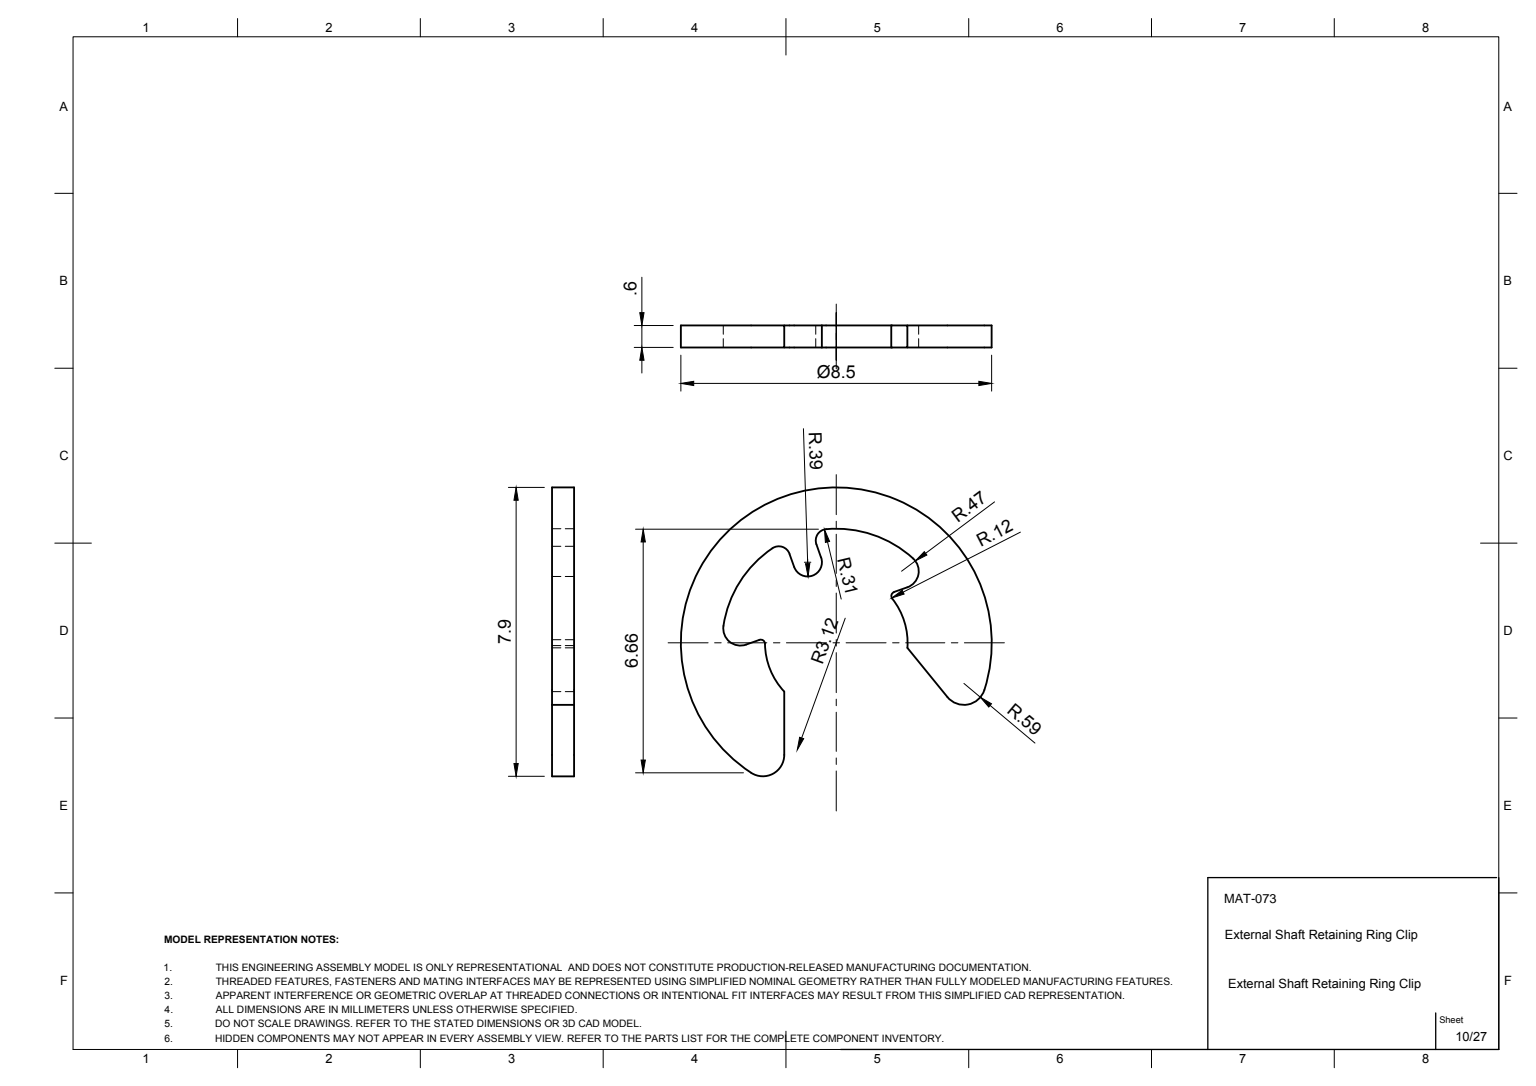
ISO-10303-21;
HEADER;
/* Generated by software containing ST-Developer
 * from STEP Tools, Inc. (www.steptools.com) 
 */

FILE_DESCRIPTION(
/* description */ ('CAx-IF Rec.Pracs.---Representation and Presentation of Product Manufa
cturing Information (PMI)---4.0---2014-10-13'),
/* implementation_level */ '2;1');

FILE_NAME(
/* name */ 'External Shaft Retaining Ring Clip.step',
/* time_stamp */ '2026-10-24T18:52:33-07:00',
/* author */ (''),
/* organization */ (''),
/* preprocessor_version */ 'ST-DEVELOPER v20.2',
/* originating_system */ 'Autodesk Translation Framework v15.17.0.0',
/* authorisation */ '');

FILE_SCHEMA (('AP242_MANAGED_MODEL_BASED_3D_ENGINEERING_MIM_LF { 1 0 10303 442 2 1 4 }'));
ENDSEC;

DATA;
#10=MECHANICAL_DESIGN_GEOMETRIC_PRESENTATION_REPRESENTATION('',(#423),#34876);
#357=SHAPE_REPRESENTATION_RELATIONSHIP('SRR','None',#34994,#390);
#390=ADVANCED_BREP_SHAPE_REPRESENTATION('',(#456),#34852);
#423=STYLED_ITEM('',(#35159),#456);
#456=MANIFOLD_SOLID_BREP('External Shaft Retaining Ring Clip',#19563);
#794=PLANE('',#20840);
#795=PLANE('',#20847);
#796=PLANE('',#20857);
#797=PLANE('',#20861);
#798=PLANE('',#20871);
#799=PLANE('',#20878);
#800=PLANE('',#20882);
#801=PLANE('',#20883);
#1677=LINE('',#30984,#3276);
#1678=LINE('',#30987,#3277);
#1679=LINE('',#30992,#3278);
#1680=LINE('',#30996,#3279);
#1681=LINE('',#30998,#3280);
#1682=LINE('',#30999,#3281);
#1683=LINE('',#31004,#3282);
#1684=LINE('',#31010,#3283);
#1685=LINE('',#31014,#3284);
#1686=LINE('',#31016,#3285);
#1687=LINE('',#31017,#3286);
#1688=LINE('',#31022,#3287);
#1689=LINE('',#31028,#3288);
#1690=LINE('',#31034,#3289);
#1691=LINE('',#31038,#3290);
#1692=LINE('',#31040,#3291);
#1693=LINE('',#31041,#3292);
#1694=LINE('',#31046,#3293);
#1695=LINE('',#31050,#3294);
#1696=LINE('',#31052,#3295);
#1697=LINE('',#31053,#3296);
#1698=LINE('',#31058,#3297);
#1699=LINE('',#31064,#3298);
#1700=LINE('',#31070,#3299);
#1701=LINE('',#31074,#3300);
#1702=LINE('',#31076,#3301);
#1703=LINE('',#31077,#3302);
#1704=LINE('',#31082,#3303);
#1705=LINE('',#31088,#3304);
#1706=LINE('',#31092,#3305);
#1707=LINE('',#31094,#3306);
#1708=LINE('',#31095,#3307);
#3276=VECTOR('',#24622,1.);
#3277=VECTOR('',#24625,1.);
#3278=VECTOR('',#24630,1.);
#3279=VECTOR('',#24635,1.);
#3280=VECTOR('',#24636,1.);
#3281=VECTOR('',#24637,1.);
#3282=VECTOR('',#24642,1.);
#3283=VECTOR('',#24649,1.);
#3284=VECTOR('',#24654,1.);
#3285=VECTOR('',#24655,1.);
#3286=VECTOR('',#24656,1.);
#3287=VECTOR('',#24661,1.);
#3288=VECTOR('',#24668,1.);
#3289=VECTOR('',#24675,1.);
#3290=VECTOR('',#24680,1.);
#3291=VECTOR('',#24681,1.);
#3292=VECTOR('',#24682,1.);
#3293=VECTOR('',#24687,1.);
#3294=VECTOR('',#24692,1.);
#3295=VECTOR('',#24693,1.);
#3296=VECTOR('',#24694,1.);
#3297=VECTOR('',#24699,1.);
#3298=VECTOR('',#24706,1.);
#3299=VECTOR('',#24713,1.);
#3300=VECTOR('',#24718,1.);
#3301=VECTOR('',#24719,1.);
#3302=VECTOR('',#24720,1.);
#3303=VECTOR('',#24725,1.);
#3304=VECTOR('',#24732,1.);
#3305=VECTOR('',#24737,1.);
#3306=VECTOR('',#24738,1.);
#3307=VECTOR('',#24739,1.);
#4468=CYLINDRICAL_SURFACE('',#20834,0.00425);
#4469=CYLINDRICAL_SURFACE('',#20837,0.000585);
#4470=CYLINDRICAL_SURFACE('',#20841,0.00195);
#4471=CYLINDRICAL_SURFACE('',#20844,0.000117);
#4472=CYLINDRICAL_SURFACE('',#20848,0.000468);
#4473=CYLINDRICAL_SURFACE('',#20851,0.00312);
#4474=CYLINDRICAL_SURFACE('',#20854,0.000312);
#4475=CYLINDRICAL_SURFACE('',#20858,0.00039);
#4476=CYLINDRICAL_SURFACE('',#20862,0.000312);
#4477=CYLINDRICAL_SURFACE('',#20865,0.00312);
#4478=CYLINDRICAL_SURFACE('',#20868,0.000468);
#4479=CYLINDRICAL_SURFACE('',#20872,0.000117);
#4480=CYLINDRICAL_SURFACE('',#20875,0.00195);
#4481=CYLINDRICAL_SURFACE('',#20879,0.000585);
#5194=FACE_OUTER_BOUND('',#6278,.T.);
#5195=FACE_OUTER_BOUND('',#6279,.T.);
#5196=FACE_OUTER_BOUND('',#6280,.T.);
#5197=FACE_OUTER_BOUND('',#6281,.T.);
#5198=FACE_OUTER_BOUND('',#6282,.T.);
#5199=FACE_OUTER_BOUND('',#6283,.T.);
#5200=FACE_OUTER_BOUND('',#6284,.T.);
#5201=FACE_OUTER_BOUND('',#6285,.T.);
#5202=FACE_OUTER_BOUND('',#6286,.T.);
#5203=FACE_OUTER_BOUND('',#6287,.T.);
#5204=FACE_OUTER_BOUND('',#6288,.T.);
#5205=FACE_OUTER_BOUND('',#6289,.T.);
#5206=FACE_OUTER_BOUND('',#6290,.T.);
#5207=FACE_OUTER_BOUND('',#6291,.T.);
#5208=FACE_OUTER_BOUND('',#6292,.T.);
#5209=FACE_OUTER_BOUND('',#6293,.T.);
#5210=FACE_OUTER_BOUND('',#6294,.T.);
#5211=FACE_OUTER_BOUND('',#6295,.T.);
#5212=FACE_OUTER_BOUND('',#6296,.T.);
#5213=FACE_OUTER_BOUND('',#6297,.T.);
#5214=FACE_OUTER_BOUND('',#6298,.T.);
#5215=FACE_OUTER_BOUND('',#6299,.T.);
#6278=EDGE_LOOP('',(#14976,#14977,#14978,#14979));
#6279=EDGE_LOOP('',(#14980,#14981,#14982,#14983));
#6280=EDGE_LOOP('',(#14984,#14985,#14986,#14987));
#6281=EDGE_LOOP('',(#14988,#14989,#14990,#14991));
#6282=EDGE_LOOP('',(#14992,#14993,#14994,#14995));
#6283=EDGE_LOOP('',(#14996,#14997,#14998,#14999));
#6284=EDGE_LOOP('',(#15000,#15001,#15002,#15003));
#6285=EDGE_LOOP('',(#15004,#15005,#15006,#15007));
#6286=EDGE_LOOP('',(#15008,#15009,#15010,#15011));
#6287=EDGE_LOOP('',(#15012,#15013,#15014,#15015));
#6288=EDGE_LOOP('',(#15016,#15017,#15018,#15019));
#6289=EDGE_LOOP('',(#15020,#15021,#15022,#15023));
#6290=EDGE_LOOP('',(#15024,#15025,#15026,#15027));
#6291=EDGE_LOOP('',(#15028,#15029,#15030,#15031));
#6292=EDGE_LOOP('',(#15032,#15033,#15034,#15035));
#6293=EDGE_LOOP('',(#15036,#15037,#15038,#15039));
#6294=EDGE_LOOP('',(#15040,#15041,#15042,#15043));
#6295=EDGE_LOOP('',(#15044,#15045,#15046,#15047));
#6296=EDGE_LOOP('',(#15048,#15049,#15050,#15051));
#6297=EDGE_LOOP('',(#15052,#15053,#15054,#15055));
#6298=EDGE_LOOP('',(#15056,#15057,#15058,#15059,#15060,#15061,#15062,#15063,
#15064,#15065,#15066,#15067,#15068,#15069,#15070,#15071,#15072,#15073,#15074,
#15075));
#6299=EDGE_LOOP('',(#15076,#15077,#15078,#15079,#15080,#15081,#15082,#15083,
#15084,#15085,#15086,#15087,#15088,#15089,#15090,#15091,#15092,#15093,#15094,
#15095));
#7376=CIRCLE('',#20835,0.00425000000001401);
#7377=CIRCLE('',#20836,0.00425000000001401);
#7378=CIRCLE('',#20838,0.000585000000012771);
#7379=CIRCLE('',#20839,0.000585000000012771);
#7380=CIRCLE('',#20842,0.00195000000001316);
#7381=CIRCLE('',#20843,0.00195000000001316);
#7382=CIRCLE('',#20845,0.00011700000001);
#7383=CIRCLE('',#20846,0.00011700000001);
#7384=CIRCLE('',#20849,0.00046800000001);
#7385=CIRCLE('',#20850,0.00046800000001);
#7386=CIRCLE('',#20852,0.00312000000001353);
#7387=CIRCLE('',#20853,0.00312000000001353);
#7388=CIRCLE('',#20855,0.000312000000012182);
#7389=CIRCLE('',#20856,0.000312000000012182);
#7390=CIRCLE('',#20859,0.00039000000001);
#7391=CIRCLE('',#20860,0.00039000000001);
#7392=CIRCLE('',#20863,0.00031200000001);
#7393=CIRCLE('',#20864,0.00031200000001);
#7394=CIRCLE('',#20866,0.00312000000001219);
#7395=CIRCLE('',#20867,0.00312000000001219);
#7396=CIRCLE('',#20869,0.00046800000001353);
#7397=CIRCLE('',#20870,0.00046800000001353);
#7398=CIRCLE('',#20873,0.000117000000012679);
#7399=CIRCLE('',#20874,0.000117000000012679);
#7400=CIRCLE('',#20876,0.00195000000001268);
#7401=CIRCLE('',#20877,0.00195000000001268);
#7402=CIRCLE('',#20880,0.000585000000014012);
#7403=CIRCLE('',#20881,0.000585000000014012);
#8792=VERTEX_POINT('',#30980);
#8793=VERTEX_POINT('',#30981);
#8794=VERTEX_POINT('',#30983);
#8795=VERTEX_POINT('',#30985);
#8796=VERTEX_POINT('',#30989);
#8797=VERTEX_POINT('',#30991);
#8798=VERTEX_POINT('',#30995);
#8799=VERTEX_POINT('',#30997);
#8800=VERTEX_POINT('',#31001);
#8801=VERTEX_POINT('',#31003);
#8802=VERTEX_POINT('',#31007);
#8803=VERTEX_POINT('',#31009);
#8804=VERTEX_POINT('',#31013);
#8805=VERTEX_POINT('',#31015);
#8806=VERTEX_POINT('',#31019);
#8807=VERTEX_POINT('',#31021);
#8808=VERTEX_POINT('',#31025);
#8809=VERTEX_POINT('',#31027);
#8810=VERTEX_POINT('',#31031);
#8811=VERTEX_POINT('',#31033);
#8812=VERTEX_POINT('',#31037);
#8813=VERTEX_POINT('',#31039);
#8814=VERTEX_POINT('',#31043);
#8815=VERTEX_POINT('',#31045);
#8816=VERTEX_POINT('',#31049);
#8817=VERTEX_POINT('',#31051);
#8818=VERTEX_POINT('',#31055);
#8819=VERTEX_POINT('',#31057);
#8820=VERTEX_POINT('',#31061);
#8821=VERTEX_POINT('',#31063);
#8822=VERTEX_POINT('',#31067);
#8823=VERTEX_POINT('',#31069);
#8824=VERTEX_POINT('',#31073);
#8825=VERTEX_POINT('',#31075);
#8826=VERTEX_POINT('',#31079);
#8827=VERTEX_POINT('',#31081);
#8828=VERTEX_POINT('',#31085);
#8829=VERTEX_POINT('',#31087);
#8830=VERTEX_POINT('',#31091);
#8831=VERTEX_POINT('',#31093);
#11046=EDGE_CURVE('',#8792,#8793,#7376,.T.);
#11047=EDGE_CURVE('',#8794,#8793,#1677,.T.);
#11048=EDGE_CURVE('',#8794,#8795,#7377,.T.);
#11049=EDGE_CURVE('',#8795,#8792,#1678,.T.);
#11050=EDGE_CURVE('',#8793,#8796,#7378,.T.);
#11051=EDGE_CURVE('',#8797,#8796,#1679,.T.);
#11052=EDGE_CURVE('',#8797,#8794,#7379,.T.);
#11053=EDGE_CURVE('',#8796,#8798,#1680,.T.);
#11054=EDGE_CURVE('',#8799,#8798,#1681,.T.);
#11055=EDGE_CURVE('',#8799,#8797,#1682,.T.);
#11056=EDGE_CURVE('',#8798,#8800,#7380,.T.);
#11057=EDGE_CURVE('',#8801,#8800,#1683,.T.);
#11058=EDGE_CURVE('',#8801,#8799,#7381,.T.);
#11059=EDGE_CURVE('',#8800,#8802,#7382,.T.);
#11060=EDGE_CURVE('',#8803,#8802,#1684,.T.);
#11061=EDGE_CURVE('',#8803,#8801,#7383,.T.);
#11062=EDGE_CURVE('',#8802,#8804,#1685,.T.);
#11063=EDGE_CURVE('',#8805,#8804,#1686,.T.);
#11064=EDGE_CURVE('',#8805,#8803,#1687,.T.);
#11065=EDGE_CURVE('',#8804,#8806,#7384,.T.);
#11066=EDGE_CURVE('',#8807,#8806,#1688,.T.);
#11067=EDGE_CURVE('',#8807,#8805,#7385,.T.);
#11068=EDGE_CURVE('',#8806,#8808,#7386,.T.);
#11069=EDGE_CURVE('',#8809,#8808,#1689,.T.);
#11070=EDGE_CURVE('',#8809,#8807,#7387,.T.);
#11071=EDGE_CURVE('',#8808,#8810,#7388,.T.);
#11072=EDGE_CURVE('',#8811,#8810,#1690,.T.);
#11073=EDGE_CURVE('',#8811,#8809,#7389,.T.);
#11074=EDGE_CURVE('',#8810,#8812,#1691,.T.);
#11075=EDGE_CURVE('',#8813,#8812,#1692,.T.);
#11076=EDGE_CURVE('',#8813,#8811,#1693,.T.);
#11077=EDGE_CURVE('',#8812,#8814,#7390,.T.);
#11078=EDGE_CURVE('',#8815,#8814,#1694,.T.);
#11079=EDGE_CURVE('',#8815,#8813,#7391,.T.);
#11080=EDGE_CURVE('',#8814,#8816,#1695,.T.);
#11081=EDGE_CURVE('',#8817,#8816,#1696,.T.);
#11082=EDGE_CURVE('',#8817,#8815,#1697,.T.);
#11083=EDGE_CURVE('',#8816,#8818,#7392,.T.);
#11084=EDGE_CURVE('',#8819,#8818,#1698,.T.);
#11085=EDGE_CURVE('',#8819,#8817,#7393,.T.);
#11086=EDGE_CURVE('',#8818,#8820,#7394,.T.);
#11087=EDGE_CURVE('',#8821,#8820,#1699,.T.);
#11088=EDGE_CURVE('',#8821,#8819,#7395,.T.);
#11089=EDGE_CURVE('',#8820,#8822,#7396,.T.);
#11090=EDGE_CURVE('',#8823,#8822,#1700,.T.);
#11091=EDGE_CURVE('',#8823,#8821,#7397,.T.);
#11092=EDGE_CURVE('',#8822,#8824,#1701,.T.);
#11093=EDGE_CURVE('',#8825,#8824,#1702,.T.);
#11094=EDGE_CURVE('',#8825,#8823,#1703,.T.);
#11095=EDGE_CURVE('',#8824,#8826,#7398,.T.);
#11096=EDGE_CURVE('',#8827,#8826,#1704,.T.);
#11097=EDGE_CURVE('',#8827,#8825,#7399,.T.);
#11098=EDGE_CURVE('',#8826,#8828,#7400,.T.);
#11099=EDGE_CURVE('',#8829,#8828,#1705,.T.);
#11100=EDGE_CURVE('',#8829,#8827,#7401,.T.);
#11101=EDGE_CURVE('',#8828,#8830,#1706,.T.);
#11102=EDGE_CURVE('',#8831,#8830,#1707,.T.);
#11103=EDGE_CURVE('',#8831,#8829,#1708,.T.);
#11104=EDGE_CURVE('',#8830,#8792,#7402,.T.);
#11105=EDGE_CURVE('',#8795,#8831,#7403,.T.);
#14976=ORIENTED_EDGE('',*,*,#11046,.T.);
#14977=ORIENTED_EDGE('',*,*,#11047,.F.);
#14978=ORIENTED_EDGE('',*,*,#11048,.T.);
#14979=ORIENTED_EDGE('',*,*,#11049,.T.);
#14980=ORIENTED_EDGE('',*,*,#11050,.T.);
#14981=ORIENTED_EDGE('',*,*,#11051,.F.);
#14982=ORIENTED_EDGE('',*,*,#11052,.T.);
#14983=ORIENTED_EDGE('',*,*,#11047,.T.);
#14984=ORIENTED_EDGE('',*,*,#11053,.T.);
#14985=ORIENTED_EDGE('',*,*,#11054,.F.);
#14986=ORIENTED_EDGE('',*,*,#11055,.T.);
#14987=ORIENTED_EDGE('',*,*,#11051,.T.);
#14988=ORIENTED_EDGE('',*,*,#11056,.T.);
#14989=ORIENTED_EDGE('',*,*,#11057,.F.);
#14990=ORIENTED_EDGE('',*,*,#11058,.T.);
#14991=ORIENTED_EDGE('',*,*,#11054,.T.);
#14992=ORIENTED_EDGE('',*,*,#11059,.T.);
#14993=ORIENTED_EDGE('',*,*,#11060,.F.);
#14994=ORIENTED_EDGE('',*,*,#11061,.T.);
#14995=ORIENTED_EDGE('',*,*,#11057,.T.);
#14996=ORIENTED_EDGE('',*,*,#11062,.T.);
#14997=ORIENTED_EDGE('',*,*,#11063,.F.);
#14998=ORIENTED_EDGE('',*,*,#11064,.T.);
#14999=ORIENTED_EDGE('',*,*,#11060,.T.);
#15000=ORIENTED_EDGE('',*,*,#11065,.T.);
#15001=ORIENTED_EDGE('',*,*,#11066,.F.);
#15002=ORIENTED_EDGE('',*,*,#11067,.T.);
#15003=ORIENTED_EDGE('',*,*,#11063,.T.);
#15004=ORIENTED_EDGE('',*,*,#11068,.T.);
#15005=ORIENTED_EDGE('',*,*,#11069,.F.);
#15006=ORIENTED_EDGE('',*,*,#11070,.T.);
#15007=ORIENTED_EDGE('',*,*,#11066,.T.);
#15008=ORIENTED_EDGE('',*,*,#11071,.T.);
#15009=ORIENTED_EDGE('',*,*,#11072,.F.);
#15010=ORIENTED_EDGE('',*,*,#11073,.T.);
#15011=ORIENTED_EDGE('',*,*,#11069,.T.);
#15012=ORIENTED_EDGE('',*,*,#11074,.T.);
#15013=ORIENTED_EDGE('',*,*,#11075,.F.);
#15014=ORIENTED_EDGE('',*,*,#11076,.T.);
#15015=ORIENTED_EDGE('',*,*,#11072,.T.);
#15016=ORIENTED_EDGE('',*,*,#11077,.T.);
#15017=ORIENTED_EDGE('',*,*,#11078,.F.);
#15018=ORIENTED_EDGE('',*,*,#11079,.T.);
#15019=ORIENTED_EDGE('',*,*,#11075,.T.);
#15020=ORIENTED_EDGE('',*,*,#11080,.T.);
#15021=ORIENTED_EDGE('',*,*,#11081,.F.);
#15022=ORIENTED_EDGE('',*,*,#11082,.T.);
#15023=ORIENTED_EDGE('',*,*,#11078,.T.);
#15024=ORIENTED_EDGE('',*,*,#11083,.T.);
#15025=ORIENTED_EDGE('',*,*,#11084,.F.);
#15026=ORIENTED_EDGE('',*,*,#11085,.T.);
#15027=ORIENTED_EDGE('',*,*,#11081,.T.);
#15028=ORIENTED_EDGE('',*,*,#11086,.T.);
#15029=ORIENTED_EDGE('',*,*,#11087,.F.);
#15030=ORIENTED_EDGE('',*,*,#11088,.T.);
#15031=ORIENTED_EDGE('',*,*,#11084,.T.);
#15032=ORIENTED_EDGE('',*,*,#11089,.T.);
#15033=ORIENTED_EDGE('',*,*,#11090,.F.);
#15034=ORIENTED_EDGE('',*,*,#11091,.T.);
#15035=ORIENTED_EDGE('',*,*,#11087,.T.);
#15036=ORIENTED_EDGE('',*,*,#11092,.T.);
#15037=ORIENTED_EDGE('',*,*,#11093,.F.);
#15038=ORIENTED_EDGE('',*,*,#11094,.T.);
#15039=ORIENTED_EDGE('',*,*,#11090,.T.);
#15040=ORIENTED_EDGE('',*,*,#11095,.T.);
#15041=ORIENTED_EDGE('',*,*,#11096,.F.);
#15042=ORIENTED_EDGE('',*,*,#11097,.T.);
#15043=ORIENTED_EDGE('',*,*,#11093,.T.);
#15044=ORIENTED_EDGE('',*,*,#11098,.T.);
#15045=ORIENTED_EDGE('',*,*,#11099,.F.);
#15046=ORIENTED_EDGE('',*,*,#11100,.T.);
#15047=ORIENTED_EDGE('',*,*,#11096,.T.);
#15048=ORIENTED_EDGE('',*,*,#11101,.T.);
#15049=ORIENTED_EDGE('',*,*,#11102,.F.);
#15050=ORIENTED_EDGE('',*,*,#11103,.T.);
#15051=ORIENTED_EDGE('',*,*,#11099,.T.);
#15052=ORIENTED_EDGE('',*,*,#11104,.T.);
#15053=ORIENTED_EDGE('',*,*,#11049,.F.);
#15054=ORIENTED_EDGE('',*,*,#11105,.T.);
#15055=ORIENTED_EDGE('',*,*,#11102,.T.);
#15056=ORIENTED_EDGE('',*,*,#11048,.F.);
#15057=ORIENTED_EDGE('',*,*,#11052,.F.);
#15058=ORIENTED_EDGE('',*,*,#11055,.F.);
#15059=ORIENTED_EDGE('',*,*,#11058,.F.);
#15060=ORIENTED_EDGE('',*,*,#11061,.F.);
#15061=ORIENTED_EDGE('',*,*,#11064,.F.);
#15062=ORIENTED_EDGE('',*,*,#11067,.F.);
#15063=ORIENTED_EDGE('',*,*,#11070,.F.);
#15064=ORIENTED_EDGE('',*,*,#11073,.F.);
#15065=ORIENTED_EDGE('',*,*,#11076,.F.);
#15066=ORIENTED_EDGE('',*,*,#11079,.F.);
#15067=ORIENTED_EDGE('',*,*,#11082,.F.);
#15068=ORIENTED_EDGE('',*,*,#11085,.F.);
#15069=ORIENTED_EDGE('',*,*,#11088,.F.);
#15070=ORIENTED_EDGE('',*,*,#11091,.F.);
#15071=ORIENTED_EDGE('',*,*,#11094,.F.);
#15072=ORIENTED_EDGE('',*,*,#11097,.F.);
#15073=ORIENTED_EDGE('',*,*,#11100,.F.);
#15074=ORIENTED_EDGE('',*,*,#11103,.F.);
#15075=ORIENTED_EDGE('',*,*,#11105,.F.);
#15076=ORIENTED_EDGE('',*,*,#11046,.F.);
#15077=ORIENTED_EDGE('',*,*,#11104,.F.);
#15078=ORIENTED_EDGE('',*,*,#11101,.F.);
#15079=ORIENTED_EDGE('',*,*,#11098,.F.);
#15080=ORIENTED_EDGE('',*,*,#11095,.F.);
#15081=ORIENTED_EDGE('',*,*,#11092,.F.);
#15082=ORIENTED_EDGE('',*,*,#11089,.F.);
#15083=ORIENTED_EDGE('',*,*,#11086,.F.);
#15084=ORIENTED_EDGE('',*,*,#11083,.F.);
#15085=ORIENTED_EDGE('',*,*,#11080,.F.);
#15086=ORIENTED_EDGE('',*,*,#11077,.F.);
#15087=ORIENTED_EDGE('',*,*,#11074,.F.);
#15088=ORIENTED_EDGE('',*,*,#11071,.F.);
#15089=ORIENTED_EDGE('',*,*,#11068,.F.);
#15090=ORIENTED_EDGE('',*,*,#11065,.F.);
#15091=ORIENTED_EDGE('',*,*,#11062,.F.);
#15092=ORIENTED_EDGE('',*,*,#11059,.F.);
#15093=ORIENTED_EDGE('',*,*,#11056,.F.);
#15094=ORIENTED_EDGE('',*,*,#11053,.F.);
#15095=ORIENTED_EDGE('',*,*,#11050,.F.);
#18910=ADVANCED_FACE('',(#5194),#4468,.T.);
#18911=ADVANCED_FACE('',(#5195),#4469,.T.);
#18912=ADVANCED_FACE('',(#5196),#794,.T.);
#18913=ADVANCED_FACE('',(#5197),#4470,.F.);
#18914=ADVANCED_FACE('',(#5198),#4471,.T.);
#18915=ADVANCED_FACE('',(#5199),#795,.T.);
#18916=ADVANCED_FACE('',(#5200),#4472,.F.);
#18917=ADVANCED_FACE('',(#5201),#4473,.F.);
#18918=ADVANCED_FACE('',(#5202),#4474,.F.);
#18919=ADVANCED_FACE('',(#5203),#796,.T.);
#18920=ADVANCED_FACE('',(#5204),#4475,.T.);
#18921=ADVANCED_FACE('',(#5205),#797,.T.);
#18922=ADVANCED_FACE('',(#5206),#4476,.F.);
#18923=ADVANCED_FACE('',(#5207),#4477,.F.);
#18924=ADVANCED_FACE('',(#5208),#4478,.F.);
#18925=ADVANCED_FACE('',(#5209),#798,.T.);
#18926=ADVANCED_FACE('',(#5210),#4479,.T.);
#18927=ADVANCED_FACE('',(#5211),#4480,.F.);
#18928=ADVANCED_FACE('',(#5212),#799,.T.);
#18929=ADVANCED_FACE('',(#5213),#4481,.T.);
#18930=ADVANCED_FACE('',(#5214),#800,.F.);
#18931=ADVANCED_FACE('',(#5215),#801,.T.);
#19563=CLOSED_SHELL('',(#18910,#18911,#18912,#18913,#18914,#18915,#18916,
#18917,#18918,#18919,#18920,#18921,#18922,#18923,#18924,#18925,#18926,#18927,
#18928,#18929,#18930,#18931));
#20833=AXIS2_PLACEMENT_3D('',#30978,#24616,#24617);
#20834=AXIS2_PLACEMENT_3D('',#30979,#24618,#24619);
#20835=AXIS2_PLACEMENT_3D('',#30982,#24620,#24621);
#20836=AXIS2_PLACEMENT_3D('',#30986,#24623,#24624);
#20837=AXIS2_PLACEMENT_3D('',#30988,#24626,#24627);
#20838=AXIS2_PLACEMENT_3D('',#30990,#24628,#24629);
#20839=AXIS2_PLACEMENT_3D('',#30993,#24631,#24632);
#20840=AXIS2_PLACEMENT_3D('',#30994,#24633,#24634);
#20841=AXIS2_PLACEMENT_3D('',#31000,#24638,#24639);
#20842=AXIS2_PLACEMENT_3D('',#31002,#24640,#24641);
#20843=AXIS2_PLACEMENT_3D('',#31005,#24643,#24644);
#20844=AXIS2_PLACEMENT_3D('',#31006,#24645,#24646);
#20845=AXIS2_PLACEMENT_3D('',#31008,#24647,#24648);
#20846=AXIS2_PLACEMENT_3D('',#31011,#24650,#24651);
#20847=AXIS2_PLACEMENT_3D('',#31012,#24652,#24653);
#20848=AXIS2_PLACEMENT_3D('',#31018,#24657,#24658);
#20849=AXIS2_PLACEMENT_3D('',#31020,#24659,#24660);
#20850=AXIS2_PLACEMENT_3D('',#31023,#24662,#24663);
#20851=AXIS2_PLACEMENT_3D('',#31024,#24664,#24665);
#20852=AXIS2_PLACEMENT_3D('',#31026,#24666,#24667);
#20853=AXIS2_PLACEMENT_3D('',#31029,#24669,#24670);
#20854=AXIS2_PLACEMENT_3D('',#31030,#24671,#24672);
#20855=AXIS2_PLACEMENT_3D('',#31032,#24673,#24674);
#20856=AXIS2_PLACEMENT_3D('',#31035,#24676,#24677);
#20857=AXIS2_PLACEMENT_3D('',#31036,#24678,#24679);
#20858=AXIS2_PLACEMENT_3D('',#31042,#24683,#24684);
#20859=AXIS2_PLACEMENT_3D('',#31044,#24685,#24686);
#20860=AXIS2_PLACEMENT_3D('',#31047,#24688,#24689);
#20861=AXIS2_PLACEMENT_3D('',#31048,#24690,#24691);
#20862=AXIS2_PLACEMENT_3D('',#31054,#24695,#24696);
#20863=AXIS2_PLACEMENT_3D('',#31056,#24697,#24698);
#20864=AXIS2_PLACEMENT_3D('',#31059,#24700,#24701);
#20865=AXIS2_PLACEMENT_3D('',#31060,#24702,#24703);
#20866=AXIS2_PLACEMENT_3D('',#31062,#24704,#24705);
#20867=AXIS2_PLACEMENT_3D('',#31065,#24707,#24708);
#20868=AXIS2_PLACEMENT_3D('',#31066,#24709,#24710);
#20869=AXIS2_PLACEMENT_3D('',#31068,#24711,#24712);
#20870=AXIS2_PLACEMENT_3D('',#31071,#24714,#24715);
#20871=AXIS2_PLACEMENT_3D('',#31072,#24716,#24717);
#20872=AXIS2_PLACEMENT_3D('',#31078,#24721,#24722);
#20873=AXIS2_PLACEMENT_3D('',#31080,#24723,#24724);
#20874=AXIS2_PLACEMENT_3D('',#31083,#24726,#24727);
#20875=AXIS2_PLACEMENT_3D('',#31084,#24728,#24729);
#20876=AXIS2_PLACEMENT_3D('',#31086,#24730,#24731);
#20877=AXIS2_PLACEMENT_3D('',#31089,#24733,#24734);
#20878=AXIS2_PLACEMENT_3D('',#31090,#24735,#24736);
#20879=AXIS2_PLACEMENT_3D('',#31096,#24740,#24741);
#20880=AXIS2_PLACEMENT_3D('',#31097,#24742,#24743);
#20881=AXIS2_PLACEMENT_3D('',#31098,#24744,#24745);
#20882=AXIS2_PLACEMENT_3D('',#31099,#24746,#24747);
#20883=AXIS2_PLACEMENT_3D('',#31100,#24748,#24749);
#24616=DIRECTION('axis',(0.,0.,1.));
#24617=DIRECTION('refdir',(1.,0.,0.));
#24618=DIRECTION('center_axis',(2.07638679158937E-16,-1.,1.20948400507518E-31));
#24619=DIRECTION('ref_axis',(0.00551570721125935,1.14527415997344E-18,0.999984788371283));
#24620=DIRECTION('center_axis',(-2.07638679158937E-16,1.,-1.20948400507518E-31));
#24621=DIRECTION('ref_axis',(0.792981602406797,1.64653652521085E-16,-0.609245581226774));
#24622=DIRECTION('',(2.07638679158937E-16,-1.,1.20948400507518E-31));
#24623=DIRECTION('center_axis',(2.07638679158937E-16,-1.,1.20948400507518E-31));
#24624=DIRECTION('ref_axis',(0.792981602406797,1.64653652521085E-16,-0.609245581226774));
#24625=DIRECTION('',(2.07638679158937E-16,-1.,1.20948400507518E-31));
#24626=DIRECTION('center_axis',(2.07638679158937E-16,-1.,1.20948400507518E-31));
#24627=DIRECTION('ref_axis',(-0.944120330982807,-1.96035898492368E-16,-0.329600971820345));
#24628=DIRECTION('center_axis',(-2.07638679158937E-16,1.,-1.20948400507518E-31));
#24629=DIRECTION('ref_axis',(-0.944120330979384,-1.96035898491658E-16,-0.329600971830149));
#24630=DIRECTION('',(2.07638679158937E-16,-1.,1.20948400507518E-31));
#24631=DIRECTION('center_axis',(2.07638679158937E-16,-1.,1.20948400507518E-31));
#24632=DIRECTION('ref_axis',(-0.944120330979384,-1.96035898491658E-16,-0.329600971830149));
#24633=DIRECTION('center_axis',(-0.944120330982807,-1.96035898492369E-16,
-0.329600971820345));
#24634=DIRECTION('ref_axis',(-0.329600971820345,-6.84379104382785E-17,0.944120330982807));
#24635=DIRECTION('',(-0.329600971820918,-6.84379104383976E-17,0.944120330982607));
#24636=DIRECTION('',(2.07638679158937E-16,-1.,1.20948400507518E-31));
#24637=DIRECTION('',(0.329600971820918,6.84379104383976E-17,-0.944120330982607));
#24638=DIRECTION('center_axis',(2.07638679158937E-16,-1.,1.20948400507518E-31));
#24639=DIRECTION('ref_axis',(-0.914294914418656,-1.89842988391623E-16,0.405049144509876));
#24640=DIRECTION('center_axis',(2.07638679158937E-16,-1.,1.20948400507518E-31));
#24641=DIRECTION('ref_axis',(-0.914294914417583,-1.898429883914E-16,0.405049144512298));
#24642=DIRECTION('',(2.07638679158937E-16,-1.,1.20948400507518E-31));
#24643=DIRECTION('center_axis',(-2.07638679158937E-16,1.,-1.20948400507518E-31));
#24644=DIRECTION('ref_axis',(-0.914294914417583,-1.898429883914E-16,0.405049144512298));
#24645=DIRECTION('center_axis',(2.07638679158937E-16,-1.,1.20948400507518E-31));
#24646=DIRECTION('ref_axis',(0.00551570721125941,1.14527415997345E-18,0.999984788371283));
#24647=DIRECTION('center_axis',(-2.07638679158937E-16,1.,-1.20948400507518E-31));
#24648=DIRECTION('ref_axis',(0.00551570721125941,1.14527415997345E-18,0.999984788371283));
#24649=DIRECTION('',(2.07638679158937E-16,-1.,1.20948400507518E-31));
#24650=DIRECTION('center_axis',(2.07638679158937E-16,-1.,1.20948400507518E-31));
#24651=DIRECTION('ref_axis',(0.00551570721125941,1.14527415997345E-18,0.999984788371283));
#24652=DIRECTION('center_axis',(0.00551570721125941,1.14527415997345E-18,
0.999984788371283));
#24653=DIRECTION('ref_axis',(0.999984788371283,2.07635520636443E-16,-0.00551570721125941));
#24654=DIRECTION('',(0.999984788371283,2.07635520636443E-16,-0.00551570721125941));
#24655=DIRECTION('',(2.07638679158937E-16,-1.,1.20948400507518E-31));
#24656=DIRECTION('',(-0.999984788371283,-2.07635520636443E-16,0.00551570721125941));
#24657=DIRECTION('center_axis',(2.07638679158937E-16,-1.,1.20948400507518E-31));
#24658=DIRECTION('ref_axis',(0.00551570721125941,1.14527415997345E-18,0.999984788371283));
#24659=DIRECTION('center_axis',(2.07638679158937E-16,-1.,1.20948400507518E-31));
#24660=DIRECTION('ref_axis',(0.00551570721125941,1.14527415997345E-18,0.999984788371283));
#24661=DIRECTION('',(2.07638679158937E-16,-1.,1.20948400507518E-31));
#24662=DIRECTION('center_axis',(-2.07638679158937E-16,1.,-1.20948400507518E-31));
#24663=DIRECTION('ref_axis',(0.00551570721125941,1.14527415997345E-18,0.999984788371283));
#24664=DIRECTION('center_axis',(2.07638679158937E-16,-1.,1.20948400507518E-31));
#24665=DIRECTION('ref_axis',(-0.884935146074078,-1.83746764872143E-16,-0.465714276400081));
#24666=DIRECTION('center_axis',(2.07638679158937E-16,-1.,1.20948400507518E-31));
#24667=DIRECTION('ref_axis',(-0.884935146073463,-1.83746764872015E-16,-0.465714276401249));
#24668=DIRECTION('',(2.07638679158937E-16,-1.,1.20948400507518E-31));
#24669=DIRECTION('center_axis',(-2.07638679158937E-16,1.,-1.20948400507518E-31));
#24670=DIRECTION('ref_axis',(-0.884935146073463,-1.83746764872015E-16,-0.465714276401249));
#24671=DIRECTION('center_axis',(2.07638679158937E-16,-1.,1.20948400507518E-31));
#24672=DIRECTION('ref_axis',(-0.255336757635762,-5.30177870962154E-17,-0.966852181152867));
#24673=DIRECTION('center_axis',(2.07638679158937E-16,-1.,1.20948400507518E-31));
#24674=DIRECTION('ref_axis',(-0.25533675765802,-5.3017787100837E-17,-0.966852181146989));
#24675=DIRECTION('',(2.07638679158937E-16,-1.,1.20948400507518E-31));
#24676=DIRECTION('center_axis',(-2.07638679158937E-16,1.,-1.20948400507518E-31));
#24677=DIRECTION('ref_axis',(-0.25533675765802,-5.3017787100837E-17,-0.966852181146989));
#24678=DIRECTION('center_axis',(0.999984788371283,2.07635520636443E-16,
-0.00551570721125978));
#24679=DIRECTION('ref_axis',(2.07638679158938E-16,-1.,1.17369458351054E-31));
#24680=DIRECTION('',(-0.00551570721225976,-1.14527416018116E-18,-0.999984788371277));
#24681=DIRECTION('',(2.07638679158937E-16,-1.,1.20948400507518E-31));
#24682=DIRECTION('',(0.00551570721225976,1.14527416018116E-18,0.999984788371277));
#24683=DIRECTION('center_axis',(2.07638679158937E-16,-1.,1.20948400507518E-31));
#24684=DIRECTION('ref_axis',(-0.999984788371283,-2.07635520636442E-16,0.00551570721125905));
#24685=DIRECTION('center_axis',(-2.07638679158937E-16,1.,-1.20948400507518E-31));
#24686=DIRECTION('ref_axis',(-0.999984788371424,-2.07635520636472E-16,0.00551570718561842));
#24687=DIRECTION('',(2.07638679158937E-16,-1.,1.20948400507518E-31));
#24688=DIRECTION('center_axis',(2.07638679158937E-16,-1.,1.20948400507518E-31));
#24689=DIRECTION('ref_axis',(-0.999984788371424,-2.07635520636472E-16,0.00551570718561842));
#24690=DIRECTION('center_axis',(-0.999984788371283,-2.07635520636443E-16,
0.00551570721125904));
#24691=DIRECTION('ref_axis',(0.00551570721125904,1.14527415997337E-18,0.999984788371283));
#24692=DIRECTION('',(0.00551570721025906,1.14527415976574E-18,0.999984788371289));
#24693=DIRECTION('',(2.07638679158937E-16,-1.,1.20948400507518E-31));
#24694=DIRECTION('',(-0.00551570721025906,-1.14527415976574E-18,-0.999984788371289));
#24695=DIRECTION('center_axis',(2.07638679158937E-16,-1.,1.20948400507518E-31));
#24696=DIRECTION('ref_axis',(-0.999984788371283,-2.07635520636442E-16,0.00551570721125908));
#24697=DIRECTION('center_axis',(2.07638679158937E-16,-1.,1.20948400507518E-31));
#24698=DIRECTION('ref_axis',(-0.99998478837146,-2.07635520636479E-16,0.00551570717920828));
#24699=DIRECTION('',(2.07638679158937E-16,-1.,1.20948400507518E-31));
#24700=DIRECTION('center_axis',(-2.07638679158937E-16,1.,-1.20948400507518E-31));
#24701=DIRECTION('ref_axis',(-0.99998478837146,-2.07635520636479E-16,0.00551570717920828));
#24702=DIRECTION('center_axis',(2.07638679158937E-16,-1.,1.20948400507518E-31));
#24703=DIRECTION('ref_axis',(0.24465563654988,5.07999732220059E-17,-0.969610034758496));
#24704=DIRECTION('center_axis',(2.07638679158937E-16,-1.,1.20948400507518E-31));
#24705=DIRECTION('ref_axis',(0.244655636552112,5.07999732224693E-17,-0.969610034757934));
#24706=DIRECTION('',(2.07638679158937E-16,-1.,1.20948400507518E-31));
#24707=DIRECTION('center_axis',(-2.07638679158937E-16,1.,-1.20948400507518E-31));
#24708=DIRECTION('ref_axis',(0.244655636552112,5.07999732224693E-17,-0.969610034757934));
#24709=DIRECTION('center_axis',(2.07638679158937E-16,-1.,1.20948400507518E-31));
#24710=DIRECTION('ref_axis',(0.879743892228186,1.82668859780403E-16,-0.475447877361127));
#24711=DIRECTION('center_axis',(2.07638679158937E-16,-1.,1.20948400507518E-31));
#24712=DIRECTION('ref_axis',(0.879743892224003,1.82668859779534E-16,-0.475447877368867));
#24713=DIRECTION('',(2.07638679158937E-16,-1.,1.20948400507518E-31));
#24714=DIRECTION('center_axis',(-2.07638679158937E-16,1.,-1.20948400507518E-31));
#24715=DIRECTION('ref_axis',(0.879743892224003,1.82668859779534E-16,-0.475447877368867));
#24716=DIRECTION('center_axis',(0.00551570721125941,1.14527415997345E-18,
0.999984788371283));
#24717=DIRECTION('ref_axis',(0.999984788371283,2.07635520636443E-16,-0.00551570721125941));
#24718=DIRECTION('',(0.999984788371283,2.07635520636443E-16,-0.00551570721125941));
#24719=DIRECTION('',(2.07638679158937E-16,-1.,1.20948400507518E-31));
#24720=DIRECTION('',(-0.999984788371283,-2.07635520636443E-16,0.00551570721125941));
#24721=DIRECTION('center_axis',(2.07638679158937E-16,-1.,1.20948400507518E-31));
#24722=DIRECTION('ref_axis',(0.945378697202868,1.962971839922E-16,-0.325974107675761));
#24723=DIRECTION('center_axis',(-2.07638679158937E-16,1.,-1.20948400507518E-31));
#24724=DIRECTION('ref_axis',(0.945378697185416,1.96297183988576E-16,-0.325974107726375));
#24725=DIRECTION('',(2.07638679158937E-16,-1.,1.20948400507518E-31));
#24726=DIRECTION('center_axis',(2.07638679158937E-16,-1.,1.20948400507518E-31));
#24727=DIRECTION('ref_axis',(0.945378697185416,1.96297183988576E-16,-0.325974107726375));
#24728=DIRECTION('center_axis',(2.07638679158937E-16,-1.,1.20948400507518E-31));
#24729=DIRECTION('ref_axis',(0.945378697202867,1.962971839922E-16,-0.325974107675763));
#24730=DIRECTION('center_axis',(2.07638679158937E-16,-1.,1.20948400507518E-31));
#24731=DIRECTION('ref_axis',(0.94537869720182,1.96297183991983E-16,-0.3259741076788));
#24732=DIRECTION('',(2.07638679158937E-16,-1.,1.20948400507518E-31));
#24733=DIRECTION('center_axis',(-2.07638679158937E-16,1.,-1.20948400507518E-31));
#24734=DIRECTION('ref_axis',(0.94537869720182,1.96297183991983E-16,-0.3259741076788));
#24735=DIRECTION('center_axis',(0.94042697538271,1.952690150139E-16,-0.339995741109396));
#24736=DIRECTION('ref_axis',(-2.07638679158937E-16,1.,-1.30537451319996E-31));
#24737=DIRECTION('',(-0.339995741109967,-7.05962666037377E-17,-0.940426975382504));
#24738=DIRECTION('',(2.07638679158937E-16,-1.,1.20948400507518E-31));
#24739=DIRECTION('',(0.339995741109967,7.05962666037377E-17,0.940426975382504));
#24740=DIRECTION('center_axis',(2.07638679158937E-16,-1.,1.20948400507518E-31));
#24741=DIRECTION('ref_axis',(-0.799654090863859,-1.66039119211012E-16,-0.600460935419362));
#24742=DIRECTION('center_axis',(-2.07638679158937E-16,1.,-1.20948400507518E-31));
#24743=DIRECTION('ref_axis',(-0.799654090861894,-1.66039119210604E-16,-0.600460935421979));
#24744=DIRECTION('center_axis',(2.07638679158937E-16,-1.,1.20948400507518E-31));
#24745=DIRECTION('ref_axis',(-0.799654090861894,-1.66039119210604E-16,-0.600460935421979));
#24746=DIRECTION('center_axis',(2.07638679158937E-16,-1.,1.20948400507518E-31));
#24747=DIRECTION('ref_axis',(0.999984788371283,2.07635520636442E-16,-0.00551570721125941));
#24748=DIRECTION('center_axis',(2.07638679158937E-16,-1.,1.20948400507518E-31));
#24749=DIRECTION('ref_axis',(0.999984788371283,2.07635520636442E-16,-0.00551570721125941));
#30978=CARTESIAN_POINT('',(0.,0.,0.));
#30979=CARTESIAN_POINT('Origin',(-4.35815392021282E-17,-0.02565,3.46944695195361E-18));
#30980=CARTESIAN_POINT('',(-0.00339852988617145,-0.02625,-0.00255195897553229));
#30981=CARTESIAN_POINT('',(0.00337017181023001,-0.02625,-0.00258929372021227));
#30982=CARTESIAN_POINT('Origin',(9.90123578286685E-15,-0.02625000000001,
-1.00514215006786E-14));
#30983=CARTESIAN_POINT('',(0.00337017181023001,-0.02565,-0.00258929372021227));
#30984=CARTESIAN_POINT('',(0.00337017181023996,-0.02565,-0.00258929372022232));
#30985=CARTESIAN_POINT('',(-0.00339852988617145,-0.02565,-0.00255195897553229));
#30986=CARTESIAN_POINT('Origin',(9.90111042199066E-15,-0.02565,-1.00514215006786E-14));
#30987=CARTESIAN_POINT('',(-0.0033985298861815,-0.02565,-0.00255195897554223));
#30988=CARTESIAN_POINT('Origin',(0.00290627757282187,-0.02565,-0.00223288505519481));
#30989=CARTESIAN_POINT('',(0.00235396717919693,-0.02625,-0.00242570162370972));
#30990=CARTESIAN_POINT('Origin',(0.00290627757283182,-0.02625000000001,
-0.00223288505520486));
#30991=CARTESIAN_POINT('',(0.00235396717919693,-0.02565,-0.00242570162370972));
#30992=CARTESIAN_POINT('',(0.00235396717920687,-0.02565,-0.00242570162371977));
#30993=CARTESIAN_POINT('Origin',(0.00290627757283182,-0.02565,-0.00223288505520486));
#30994=CARTESIAN_POINT('Origin',(0.00235396717919693,-0.02565,-0.00242570162370972));
#30995=CARTESIAN_POINT('',(0.00178287508311634,-0.02625,-0.000789845831794254));
#30996=CARTESIAN_POINT('',(0.00178287508312629,-0.02625000000001,-0.000789845831804309));
#30997=CARTESIAN_POINT('',(0.00178287508311634,-0.02565,-0.000789845831794254));
#30998=CARTESIAN_POINT('',(0.00178287508312629,-0.02565,-0.000789845831804309));
#30999=CARTESIAN_POINT('',(0.00178287508312629,-0.02565,-0.000789845831804309));
#31000=CARTESIAN_POINT('Origin',(-4.35815392021282E-17,-0.02565,3.46944695195361E-18));
#31001=CARTESIAN_POINT('',(0.00185038829705699,-0.02625,0.000615274857372195));
#31002=CARTESIAN_POINT('Origin',(9.90123578286685E-15,-0.02625000000001,
-1.00514215006786E-14));
#31003=CARTESIAN_POINT('',(0.00185038829705699,-0.02565,0.000615274857372195));
#31004=CARTESIAN_POINT('',(0.00185038829706693,-0.02565,0.00061527485736214));
#31005=CARTESIAN_POINT('Origin',(9.90111042199066E-15,-0.02565,-1.00514215006786E-14));
#31006=CARTESIAN_POINT('Origin',(0.00196141159488042,-0.02565,0.000652191348814524));
#31007=CARTESIAN_POINT('',(0.00196205693262413,-0.02625,0.000769189569053964));
#31008=CARTESIAN_POINT('Origin',(0.00196141159489036,-0.02625000000001,
0.000652191348804469));
#31009=CARTESIAN_POINT('',(0.00196205693262413,-0.02565,0.000769189569053964));
#31010=CARTESIAN_POINT('',(0.00196205693263408,-0.02565,0.000769189569043909));
#31011=CARTESIAN_POINT('Origin',(0.00196141159489036,-0.02565,0.000652191348804469));
#31012=CARTESIAN_POINT('Origin',(0.00196205693262413,-0.02565,0.000769189569053964));
#31013=CARTESIAN_POINT('',(0.00234426665641354,-0.02625,0.000767081380055257));
#31014=CARTESIAN_POINT('',(0.00234426665642348,-0.02625000000001,0.000767081380045202));
#31015=CARTESIAN_POINT('',(0.00234426665641354,-0.02565,0.000767081380055257));
#31016=CARTESIAN_POINT('',(0.00234426665642348,-0.02565,0.000767081380045202));
#31017=CARTESIAN_POINT('',(0.00234426665642348,-0.02565,0.000767081380045202));
#31018=CARTESIAN_POINT('Origin',(0.00234684800738841,-0.02565,0.00123507426101302));
#31019=CARTESIAN_POINT('',(0.00276099765575108,-0.02625,0.00145302854236826));
#31020=CARTESIAN_POINT('Origin',(0.00234684800739835,-0.02625000000001,
0.00123507426100296));
#31021=CARTESIAN_POINT('',(0.00276099765575108,-0.02565,0.00145302854236826));
#31022=CARTESIAN_POINT('',(0.00276099765576102,-0.02565,0.0014530285423582));
#31023=CARTESIAN_POINT('Origin',(0.00234684800739835,-0.02565,0.00123507426100296));
#31024=CARTESIAN_POINT('Origin',(-4.35815392021282E-17,-0.02565,3.46944695195361E-18));
#31025=CARTESIAN_POINT('',(0.000796650683823533,-0.02625,0.00301657880519694));
#31026=CARTESIAN_POINT('Origin',(9.90123578286685E-15,-0.02625000000001,
-1.00514215006786E-14));
#31027=CARTESIAN_POINT('',(0.000796650683823533,-0.02565,0.00301657880519694));
#31028=CARTESIAN_POINT('',(0.000796650683833588,-0.02565,0.00301657880520689));
#31029=CARTESIAN_POINT('Origin',(9.90111042199066E-15,-0.02565,-1.00514215006786E-14));
#31030=CARTESIAN_POINT('Origin',(0.000716985615441175,-0.02565,0.00271492092467725));
#31031=CARTESIAN_POINT('',(0.000404990361469335,-0.02625,0.00271664182532716));
#31032=CARTESIAN_POINT('Origin',(0.00071698561545123,-0.02625000000001,
0.0027149209246872));
#31033=CARTESIAN_POINT('',(0.000404990361469334,-0.02565,0.00271664182532716));
#31034=CARTESIAN_POINT('',(0.000404990361479389,-0.02565,0.00271664182533711));
#31035=CARTESIAN_POINT('Origin',(0.00071698561545123,-0.02565,0.0027149209246872));
#31036=CARTESIAN_POINT('Origin',(0.000404990361469334,-0.02565,0.00271664182532716));
#31037=CARTESIAN_POINT('',(0.000402900822339103,-0.02625,0.00233781327897642));
#31038=CARTESIAN_POINT('',(0.000402900822349048,-0.02625000000001,0.00233781327896636));
#31039=CARTESIAN_POINT('',(0.000402900822339103,-0.02565,0.00233781327897642));
#31040=CARTESIAN_POINT('',(0.000402900822349048,-0.02565,0.00233781327896636));
#31041=CARTESIAN_POINT('',(0.000402900822349048,-0.02565,0.00233781327896636));
#31042=CARTESIAN_POINT('Origin',(1.29067548743032E-5,-0.02565,0.00233996440478881));
#31043=CARTESIAN_POINT('',(-0.000377087312590497,-0.02625,0.0023421155306012));
#31044=CARTESIAN_POINT('Origin',(1.29067548742481E-5,-0.02625000000001,
0.00233996440477881));
#31045=CARTESIAN_POINT('',(-0.000377087312590497,-0.02565,0.0023421155306012));
#31046=CARTESIAN_POINT('',(-0.000377087312600552,-0.02565,0.00234211553059125));
#31047=CARTESIAN_POINT('Origin',(1.2906754874248E-5,-0.02565,0.00233996440477881));
#31048=CARTESIAN_POINT('Origin',(-0.000377087312590497,-0.02565,0.0023421155306012));
#31049=CARTESIAN_POINT('',(-0.000374997773460266,-0.02625,0.00272094407695195));
#31050=CARTESIAN_POINT('',(-0.000374997773470211,-0.02625000000001,0.00272094407696201));
#31051=CARTESIAN_POINT('',(-0.000374997773460266,-0.02565,0.00272094407695195));
#31052=CARTESIAN_POINT('',(-0.000374997773470211,-0.02565,0.00272094407696201));
#31053=CARTESIAN_POINT('',(-0.000374997773470211,-0.02565,0.00272094407696201));
#31054=CARTESIAN_POINT('Origin',(-0.000686993027432106,-0.02565,0.00272266497760186));
#31055=CARTESIAN_POINT('',(-0.000763325586035669,-0.02625,0.00302518330844651));
#31056=CARTESIAN_POINT('Origin',(-0.000686993027442051,-0.02625000000001,
0.00272266497761192));
#31057=CARTESIAN_POINT('',(-0.000763325586035669,-0.02565,0.00302518330844651));
#31058=CARTESIAN_POINT('',(-0.000763325586045614,-0.02565,0.00302518330845656));
#31059=CARTESIAN_POINT('Origin',(-0.000686993027442051,-0.02565,0.00272266497761192));
#31060=CARTESIAN_POINT('Origin',(-4.35815392021282E-17,-0.02565,3.46944695195361E-18));
#31061=CARTESIAN_POINT('',(-0.00274480094375199,-0.02625,0.00148339737736672));
#31062=CARTESIAN_POINT('Origin',(9.90123578286685E-15,-0.02625000000001,
-1.00514215006786E-14));
#31063=CARTESIAN_POINT('',(-0.00274480094375199,-0.02565,0.00148339737736672));
#31064=CARTESIAN_POINT('',(-0.00274480094376204,-0.02565,0.00148339737735678));
#31065=CARTESIAN_POINT('Origin',(9.90111042199066E-15,-0.02565,-1.00514215006786E-14));
#31066=CARTESIAN_POINT('Origin',(-0.00233308080218919,-0.02565,0.00126088777076171));
#31067=CARTESIAN_POINT('',(-0.00233566215316406,-0.02625,0.000792894889803951));
#31068=CARTESIAN_POINT('Origin',(-0.00233308080219925,-0.02625000000001,
0.00126088777075177));
#31069=CARTESIAN_POINT('',(-0.00233566215316406,-0.02565,0.000792894889803951));
#31070=CARTESIAN_POINT('',(-0.00233566215317412,-0.02565,0.000792894889794006));
#31071=CARTESIAN_POINT('Origin',(-0.00233308080219925,-0.02565,0.00126088777075177));
#31072=CARTESIAN_POINT('Origin',(-0.00233566215316406,-0.02565,0.000792894889803951));
#31073=CARTESIAN_POINT('',(-0.00195345242937466,-0.02625,0.000790786700805244));
#31074=CARTESIAN_POINT('',(-0.00195345242938471,-0.02625000000001,0.000790786700795299));
#31075=CARTESIAN_POINT('',(-0.00195345242937466,-0.02565,0.000790786700805244));
#31076=CARTESIAN_POINT('',(-0.00195345242938471,-0.02565,0.000790786700795299));
#31077=CARTESIAN_POINT('',(-0.00195345242938471,-0.02565,0.000790786700795299));
#31078=CARTESIAN_POINT('Origin',(-0.00195409776711838,-0.02565,0.000673788480565804));
#31079=CARTESIAN_POINT('',(-0.00184348845954563,-0.02625,0.000635649509967742));
#31080=CARTESIAN_POINT('Origin',(-0.00195409776712843,-0.02625000000001,
0.000673788480555859));
#31081=CARTESIAN_POINT('',(-0.00184348845954563,-0.02565,0.000635649509967742));
#31082=CARTESIAN_POINT('',(-0.00184348845955569,-0.02565,0.000635649509957798));
#31083=CARTESIAN_POINT('Origin',(-0.00195409776712843,-0.02565,0.000673788480555859));
#31084=CARTESIAN_POINT('Origin',(-4.35815392021282E-17,-0.02565,3.46944695195361E-18));
#31085=CARTESIAN_POINT('',(-0.00179147958636599,-0.02625,-0.000770130438064942));
#31086=CARTESIAN_POINT('Origin',(9.90123578286685E-15,-0.02625000000001,
-1.00514215006786E-14));
#31087=CARTESIAN_POINT('',(-0.00179147958636599,-0.02565,-0.000770130438064942));
#31088=CARTESIAN_POINT('',(-0.00179147958637604,-0.02565,-0.000770130438074886));
#31089=CARTESIAN_POINT('Origin',(9.90111042199066E-15,-0.02565,-1.00514215006786E-14));
#31090=CARTESIAN_POINT('Origin',(-0.00179147958636599,-0.02565,-0.000770130438064942));
#31091=CARTESIAN_POINT('',(-0.0023805824624172,-0.02625,-0.00239958683686096));
#31092=CARTESIAN_POINT('',(-0.00238058246242725,-0.02625000000001,-0.00239958683687091));
#31093=CARTESIAN_POINT('',(-0.0023805824624172,-0.02565,-0.00239958683686096));
#31094=CARTESIAN_POINT('',(-0.00238058246242725,-0.02565,-0.00239958683687091));
#31095=CARTESIAN_POINT('',(-0.00238058246242725,-0.02565,-0.00239958683687091));
#31096=CARTESIAN_POINT('Origin',(-0.00293073224301609,-0.02565,-0.00220068932831195));
#31097=CARTESIAN_POINT('Origin',(-0.00293073224302614,-0.02625000000001,
-0.0022006893283219));
#31098=CARTESIAN_POINT('Origin',(-0.00293073224302614,-0.02565,-0.0022006893283219));
#31099=CARTESIAN_POINT('Origin',(5.35383428478025E-6,-0.02565,0.000970637606244856));
#31100=CARTESIAN_POINT('Origin',(5.35383428478008E-6,-0.02625,0.000970637606244856));
#34817=UNCERTAINTY_MEASURE_WITH_UNIT(LENGTH_MEASURE(1.E-5),#34877,
'DISTANCE_ACCURACY_VALUE',
'Maximum model space distance between geometric entities at asserted c
onnectivities');
#34841=UNCERTAINTY_MEASURE_WITH_UNIT(LENGTH_MEASURE(1.E-5),#34877,
'DISTANCE_ACCURACY_VALUE',
'Maximum model space distance between geometric entities at asserted c
onnectivities');
#34852=(
GEOMETRIC_REPRESENTATION_CONTEXT(3)
GLOBAL_UNCERTAINTY_ASSIGNED_CONTEXT((#34817))
GLOBAL_UNIT_ASSIGNED_CONTEXT((#34877,#34878,#34879))
REPRESENTATION_CONTEXT('','3D')
);
#34876=(
GEOMETRIC_REPRESENTATION_CONTEXT(3)
GLOBAL_UNCERTAINTY_ASSIGNED_CONTEXT((#34841))
GLOBAL_UNIT_ASSIGNED_CONTEXT((#34877,#34878,#34879))
REPRESENTATION_CONTEXT('','3D')
);
#34877=(
LENGTH_UNIT()
NAMED_UNIT(*)
SI_UNIT($,.METRE.)
);
#34878=(
NAMED_UNIT(*)
PLANE_ANGLE_UNIT()
SI_UNIT($,.RADIAN.)
);
#34879=(
NAMED_UNIT(*)
SI_UNIT($,.STERADIAN.)
SOLID_ANGLE_UNIT()
);
#34890=SHAPE_DEFINITION_REPRESENTATION(#34924,#34994);
#34924=PRODUCT_DEFINITION_SHAPE('',$,#35029);
#34994=SHAPE_REPRESENTATION('',(#20833),#34852);
#35018=PRODUCT_DEFINITION_CONTEXT('part definition',#35122,'design');
#35029=PRODUCT_DEFINITION('External Shaft Retaining Ring Clip',
'External Shaft Retaining Ring Clip',#35063,#35018);
#35063=PRODUCT_DEFINITION_FORMATION('',$,#35134);
#35122=APPLICATION_CONTEXT('Managed model based 3d engineering');
#35123=PRODUCT_CONTEXT('part definition',#35122,'mechanical');
#35134=PRODUCT('External Shaft Retaining Ring Clip',
'External Shaft Retaining Ring Clip',
'LEGAL AND USAGE DISCLAIMER: this Data/Model is provided \X2\201C\X0\A
S IS\X2\201D\X0\ for informational and representational only. It is a 
geometric approximation and is NOT engineered, certified, or guarantee
d for dimensional accuracy, exact tolerances, or production-level prec
ision. Vendor disclaims all implied warranties including fitness for a
 particular purpose. DO NOT USE FOR DIRECT PHYSICAL MANUFACTURING, AUT
OMATED PRODUCTION, OR SAFETY-CRITICAL SYSTEMS without independent engi
neering verification and resolution of any design discrepancies.',(#35123));
#35159=PRESENTATION_STYLE_ASSIGNMENT((#35168));
#35168=SURFACE_STYLE_USAGE(.BOTH.,#35177);
#35177=SURFACE_SIDE_STYLE('',(#35186));
#35186=SURFACE_STYLE_FILL_AREA(#35195);
#35195=FILL_AREA_STYLE('Paint - Enamel Glossy (White)',(#35204));
#35204=FILL_AREA_STYLE_COLOUR('Paint - Enamel Glossy (White)',#35213);
#35213=COLOUR_RGB('Paint - Enamel Glossy (White)',0.964705882352941,0.964705882352941,
0.952941176470588);
ENDSEC;
END-ISO-10303-21;
